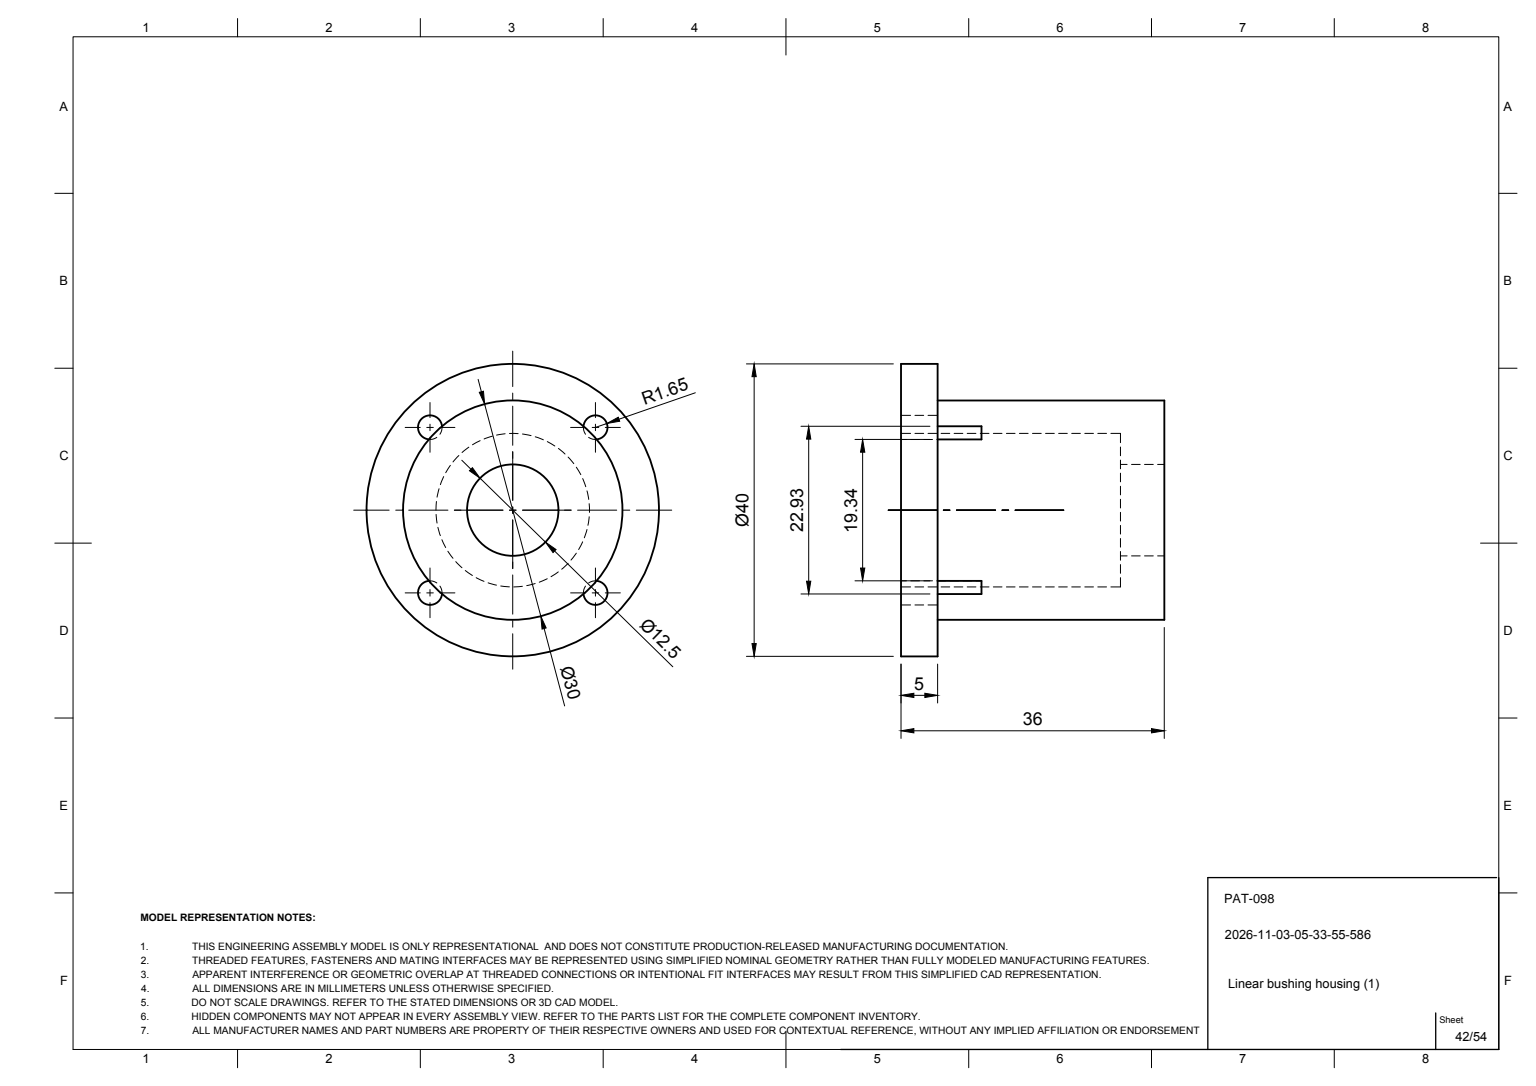
ISO-10303-21;
HEADER;
/* Generated by software containing ST-Developer
 * from STEP Tools, Inc. (www.steptools.com) 
 */

FILE_DESCRIPTION(
/* description */ ('Spring compression tester'),
/* implementation_level */ '2;1');

FILE_NAME(
/* name */ 'Linear bushing housing (1).step',
/* time_stamp */ '2026-10-28T03:24:11-07:00',
/* author */ (''),
/* organization */ (''),
/* preprocessor_version */ 'ST-DEVELOPER v20.2',
/* originating_system */ 'Autodesk Translation Framework v15.17.0.0',
/* authorisation */ '');

FILE_SCHEMA (('AUTOMOTIVE_DESIGN { 1 0 10303 214 3 1 1 }'));
ENDSEC;

DATA;
#10=MECHANICAL_DESIGN_GEOMETRIC_PRESENTATION_REPRESENTATION('',(#1160),#43521);
#1025=SHAPE_REPRESENTATION_RELATIONSHIP('SRR','None',#43840,#1085);
#1085=ADVANCED_BREP_SHAPE_REPRESENTATION('',(#1231),#43500);
#1160=STYLED_ITEM('',(#44181),#1231);
#1231=MANIFOLD_SOLID_BREP('Body1',#18601);
#1521=FACE_BOUND('',#4194,.T.);
#1522=FACE_BOUND('',#4196,.T.);
#1523=FACE_BOUND('',#4200,.T.);
#1524=FACE_BOUND('',#4201,.T.);
#1525=FACE_BOUND('',#4202,.T.);
#1526=FACE_BOUND('',#4203,.T.);
#1527=FACE_BOUND('',#4204,.T.);
#1528=FACE_BOUND('',#4206,.T.);
#2038=PLANE('',#20538);
#2039=PLANE('',#20545);
#2040=PLANE('',#20552);
#2041=PLANE('',#20559);
#2042=PLANE('',#20576);
#2043=PLANE('',#20578);
#2044=PLANE('',#20584);
#2045=PLANE('',#20585);
#2862=FACE_OUTER_BOUND('',#4183,.T.);
#2863=FACE_OUTER_BOUND('',#4184,.T.);
#2864=FACE_OUTER_BOUND('',#4185,.T.);
#2865=FACE_OUTER_BOUND('',#4186,.T.);
#2866=FACE_OUTER_BOUND('',#4187,.T.);
#2867=FACE_OUTER_BOUND('',#4188,.T.);
#2868=FACE_OUTER_BOUND('',#4189,.T.);
#2869=FACE_OUTER_BOUND('',#4190,.T.);
#2870=FACE_OUTER_BOUND('',#4191,.T.);
#2871=FACE_OUTER_BOUND('',#4192,.T.);
#2872=FACE_OUTER_BOUND('',#4193,.T.);
#2873=FACE_OUTER_BOUND('',#4195,.T.);
#2874=FACE_OUTER_BOUND('',#4197,.T.);
#2875=FACE_OUTER_BOUND('',#4198,.T.);
#2876=FACE_OUTER_BOUND('',#4199,.T.);
#2877=FACE_OUTER_BOUND('',#4205,.T.);
#4183=EDGE_LOOP('',(#15357,#15358));
#4184=EDGE_LOOP('',(#15359,#15360,#15361,#15362,#15363,#15364,#15365,#15366));
#4185=EDGE_LOOP('',(#15367,#15368));
#4186=EDGE_LOOP('',(#15369,#15370,#15371,#15372,#15373,#15374,#15375,#15376));
#4187=EDGE_LOOP('',(#15377,#15378,#15379));
#4188=EDGE_LOOP('',(#15380,#15381,#15382,#15383,#15384,#15385,#15386,#15387));
#4189=EDGE_LOOP('',(#15388,#15389,#15390));
#4190=EDGE_LOOP('',(#15391,#15392,#15393,#15394,#15395,#15396,#15397,#15398));
#4191=EDGE_LOOP('',(#15399,#15400,#15401,#15402,#15403,#15404,#15405,#15406,
#15407,#15408,#15409,#15410,#15411,#15412,#15413,#15414,#15415,#15416,#15417,
#15418));
#4192=EDGE_LOOP('',(#15419,#15420,#15421,#15422));
#4193=EDGE_LOOP('',(#15423));
#4194=EDGE_LOOP('',(#15424));
#4195=EDGE_LOOP('',(#15425));
#4196=EDGE_LOOP('',(#15426,#15427,#15428,#15429,#15430,#15431,#15432,#15433,
#15434,#15435,#15436));
#4197=EDGE_LOOP('',(#15437,#15438,#15439,#15440));
#4198=EDGE_LOOP('',(#15441,#15442,#15443,#15444));
#4199=EDGE_LOOP('',(#15445));
#4200=EDGE_LOOP('',(#15446));
#4201=EDGE_LOOP('',(#15447));
#4202=EDGE_LOOP('',(#15448));
#4203=EDGE_LOOP('',(#15449));
#4204=EDGE_LOOP('',(#15450));
#4205=EDGE_LOOP('',(#15451));
#4206=EDGE_LOOP('',(#15452));
#5639=LINE('',#30468,#7071);
#5640=LINE('',#30472,#7072);
#5641=LINE('',#30476,#7073);
#5642=LINE('',#30484,#7074);
#5643=LINE('',#30488,#7075);
#5644=LINE('',#30492,#7076);
#5645=LINE('',#30502,#7077);
#5646=LINE('',#30505,#7078);
#5647=LINE('',#30507,#7079);
#5648=LINE('',#30518,#7080);
#5649=LINE('',#30521,#7081);
#5650=LINE('',#30523,#7082);
#5651=LINE('',#30529,#7083);
#5652=LINE('',#30539,#7084);
#5653=LINE('',#30550,#7085);
#5654=LINE('',#30553,#7086);
#7071=VECTOR('',#24745,1.);
#7072=VECTOR('',#24748,0.165);
#7073=VECTOR('',#24753,1.);
#7074=VECTOR('',#24762,1.);
#7075=VECTOR('',#24765,0.165);
#7076=VECTOR('',#24770,1.);
#7077=VECTOR('',#24781,1.);
#7078=VECTOR('',#24784,1.);
#7079=VECTOR('',#24785,0.165);
#7080=VECTOR('',#24798,1.);
#7081=VECTOR('',#24801,1.);
#7082=VECTOR('',#24802,0.165);
#7083=VECTOR('',#24809,1.5);
#7084=VECTOR('',#24824,1.05);
#7085=VECTOR('',#24839,2.);
#7086=VECTOR('',#24842,0.625);
#7973=CIRCLE('',#20539,1.5);
#7974=CIRCLE('',#20540,0.165);
#7975=CIRCLE('',#20542,0.165);
#7976=CIRCLE('',#20543,0.165);
#7977=CIRCLE('',#20544,0.165);
#7978=CIRCLE('',#20546,1.5);
#7979=CIRCLE('',#20547,0.165);
#7980=CIRCLE('',#20549,0.165);
#7981=CIRCLE('',#20550,0.165);
#7982=CIRCLE('',#20551,0.165);
#7983=CIRCLE('',#20553,1.5);
#7984=CIRCLE('',#20554,0.165);
#7985=CIRCLE('',#20555,0.165);
#7986=CIRCLE('',#20557,0.165);
#7987=CIRCLE('',#20558,0.165);
#7988=CIRCLE('',#20560,1.5);
#7989=CIRCLE('',#20561,0.165);
#7990=CIRCLE('',#20562,0.165);
#7991=CIRCLE('',#20564,0.165);
#7992=CIRCLE('',#20565,0.165);
#7993=CIRCLE('',#20567,1.5);
#7994=CIRCLE('',#20568,1.5);
#7995=CIRCLE('',#20569,1.5);
#7996=CIRCLE('',#20570,1.5);
#7997=CIRCLE('',#20571,1.5);
#7998=CIRCLE('',#20572,1.5);
#7999=CIRCLE('',#20574,1.05);
#8000=CIRCLE('',#20575,1.05);
#8001=CIRCLE('',#20577,0.625);
#8002=CIRCLE('',#20579,2.);
#8003=CIRCLE('',#20581,2.);
#8004=CIRCLE('',#20583,0.625);
#9194=VERTEX_POINT('',#30462);
#9195=VERTEX_POINT('',#30463);
#9196=VERTEX_POINT('',#30467);
#9197=VERTEX_POINT('',#30469);
#9198=VERTEX_POINT('',#30471);
#9199=VERTEX_POINT('',#30474);
#9200=VERTEX_POINT('',#30478);
#9201=VERTEX_POINT('',#30479);
#9202=VERTEX_POINT('',#30483);
#9203=VERTEX_POINT('',#30485);
#9204=VERTEX_POINT('',#30487);
#9205=VERTEX_POINT('',#30490);
#9206=VERTEX_POINT('',#30494);
#9207=VERTEX_POINT('',#30495);
#9208=VERTEX_POINT('',#30497);
#9209=VERTEX_POINT('',#30501);
#9210=VERTEX_POINT('',#30503);
#9211=VERTEX_POINT('',#30506);
#9212=VERTEX_POINT('',#30510);
#9213=VERTEX_POINT('',#30511);
#9214=VERTEX_POINT('',#30513);
#9215=VERTEX_POINT('',#30517);
#9216=VERTEX_POINT('',#30519);
#9217=VERTEX_POINT('',#30522);
#9218=VERTEX_POINT('',#30526);
#9219=VERTEX_POINT('',#30528);
#9220=VERTEX_POINT('',#30536);
#9221=VERTEX_POINT('',#30538);
#9222=VERTEX_POINT('',#30542);
#9223=VERTEX_POINT('',#30545);
#9224=VERTEX_POINT('',#30548);
#9225=VERTEX_POINT('',#30552);
#11343=EDGE_CURVE('',#9194,#9195,#7973,.T.);
#11344=EDGE_CURVE('',#9194,#9195,#7974,.T.);
#11345=EDGE_CURVE('',#9196,#9194,#5639,.T.);
#11346=EDGE_CURVE('',#9197,#9196,#7975,.T.);
#11347=EDGE_CURVE('',#9197,#9198,#5640,.T.);
#11348=EDGE_CURVE('',#9198,#9198,#7976,.T.);
#11349=EDGE_CURVE('',#9199,#9197,#7977,.T.);
#11350=EDGE_CURVE('',#9195,#9199,#5641,.T.);
#11351=EDGE_CURVE('',#9200,#9201,#7978,.T.);
#11352=EDGE_CURVE('',#9200,#9201,#7979,.T.);
#11353=EDGE_CURVE('',#9202,#9200,#5642,.T.);
#11354=EDGE_CURVE('',#9203,#9202,#7980,.T.);
#11355=EDGE_CURVE('',#9203,#9204,#5643,.T.);
#11356=EDGE_CURVE('',#9204,#9204,#7981,.T.);
#11357=EDGE_CURVE('',#9205,#9203,#7982,.T.);
#11358=EDGE_CURVE('',#9201,#9205,#5644,.T.);
#11359=EDGE_CURVE('',#9206,#9207,#7983,.T.);
#11360=EDGE_CURVE('',#9206,#9208,#7984,.T.);
#11361=EDGE_CURVE('',#9208,#9207,#7985,.T.);
#11362=EDGE_CURVE('',#9209,#9206,#5645,.T.);
#11363=EDGE_CURVE('',#9210,#9209,#7986,.T.);
#11364=EDGE_CURVE('',#9207,#9210,#5646,.T.);
#11365=EDGE_CURVE('',#9208,#9211,#5647,.T.);
#11366=EDGE_CURVE('',#9211,#9211,#7987,.T.);
#11367=EDGE_CURVE('',#9212,#9213,#7988,.T.);
#11368=EDGE_CURVE('',#9212,#9214,#7989,.T.);
#11369=EDGE_CURVE('',#9214,#9213,#7990,.T.);
#11370=EDGE_CURVE('',#9215,#9212,#5648,.T.);
#11371=EDGE_CURVE('',#9216,#9215,#7991,.T.);
#11372=EDGE_CURVE('',#9213,#9216,#5649,.T.);
#11373=EDGE_CURVE('',#9214,#9217,#5650,.T.);
#11374=EDGE_CURVE('',#9217,#9217,#7992,.T.);
#11375=EDGE_CURVE('',#9199,#9218,#7993,.T.);
#11376=EDGE_CURVE('',#9218,#9219,#5651,.T.);
#11377=EDGE_CURVE('',#9219,#9219,#7994,.T.);
#11378=EDGE_CURVE('',#9218,#9202,#7995,.T.);
#11379=EDGE_CURVE('',#9205,#9209,#7996,.T.);
#11380=EDGE_CURVE('',#9210,#9215,#7997,.T.);
#11381=EDGE_CURVE('',#9216,#9196,#7998,.T.);
#11382=EDGE_CURVE('',#9220,#9220,#7999,.T.);
#11383=EDGE_CURVE('',#9220,#9221,#5652,.T.);
#11384=EDGE_CURVE('',#9221,#9221,#8000,.T.);
#11385=EDGE_CURVE('',#9222,#9222,#8001,.T.);
#11386=EDGE_CURVE('',#9223,#9223,#8002,.T.);
#11387=EDGE_CURVE('',#9224,#9224,#8003,.T.);
#11388=EDGE_CURVE('',#9224,#9223,#5653,.T.);
#11389=EDGE_CURVE('',#9222,#9225,#5654,.T.);
#11390=EDGE_CURVE('',#9225,#9225,#8004,.T.);
#15357=ORIENTED_EDGE('',*,*,#11343,.F.);
#15358=ORIENTED_EDGE('',*,*,#11344,.T.);
#15359=ORIENTED_EDGE('',*,*,#11345,.F.);
#15360=ORIENTED_EDGE('',*,*,#11346,.F.);
#15361=ORIENTED_EDGE('',*,*,#11347,.T.);
#15362=ORIENTED_EDGE('',*,*,#11348,.F.);
#15363=ORIENTED_EDGE('',*,*,#11347,.F.);
#15364=ORIENTED_EDGE('',*,*,#11349,.F.);
#15365=ORIENTED_EDGE('',*,*,#11350,.F.);
#15366=ORIENTED_EDGE('',*,*,#11344,.F.);
#15367=ORIENTED_EDGE('',*,*,#11351,.F.);
#15368=ORIENTED_EDGE('',*,*,#11352,.T.);
#15369=ORIENTED_EDGE('',*,*,#11353,.F.);
#15370=ORIENTED_EDGE('',*,*,#11354,.F.);
#15371=ORIENTED_EDGE('',*,*,#11355,.T.);
#15372=ORIENTED_EDGE('',*,*,#11356,.F.);
#15373=ORIENTED_EDGE('',*,*,#11355,.F.);
#15374=ORIENTED_EDGE('',*,*,#11357,.F.);
#15375=ORIENTED_EDGE('',*,*,#11358,.F.);
#15376=ORIENTED_EDGE('',*,*,#11352,.F.);
#15377=ORIENTED_EDGE('',*,*,#11359,.F.);
#15378=ORIENTED_EDGE('',*,*,#11360,.T.);
#15379=ORIENTED_EDGE('',*,*,#11361,.T.);
#15380=ORIENTED_EDGE('',*,*,#11362,.F.);
#15381=ORIENTED_EDGE('',*,*,#11363,.F.);
#15382=ORIENTED_EDGE('',*,*,#11364,.F.);
#15383=ORIENTED_EDGE('',*,*,#11361,.F.);
#15384=ORIENTED_EDGE('',*,*,#11365,.T.);
#15385=ORIENTED_EDGE('',*,*,#11366,.F.);
#15386=ORIENTED_EDGE('',*,*,#11365,.F.);
#15387=ORIENTED_EDGE('',*,*,#11360,.F.);
#15388=ORIENTED_EDGE('',*,*,#11367,.F.);
#15389=ORIENTED_EDGE('',*,*,#11368,.T.);
#15390=ORIENTED_EDGE('',*,*,#11369,.T.);
#15391=ORIENTED_EDGE('',*,*,#11370,.F.);
#15392=ORIENTED_EDGE('',*,*,#11371,.F.);
#15393=ORIENTED_EDGE('',*,*,#11372,.F.);
#15394=ORIENTED_EDGE('',*,*,#11369,.F.);
#15395=ORIENTED_EDGE('',*,*,#11373,.T.);
#15396=ORIENTED_EDGE('',*,*,#11374,.F.);
#15397=ORIENTED_EDGE('',*,*,#11373,.F.);
#15398=ORIENTED_EDGE('',*,*,#11368,.F.);
#15399=ORIENTED_EDGE('',*,*,#11345,.T.);
#15400=ORIENTED_EDGE('',*,*,#11343,.T.);
#15401=ORIENTED_EDGE('',*,*,#11350,.T.);
#15402=ORIENTED_EDGE('',*,*,#11375,.T.);
#15403=ORIENTED_EDGE('',*,*,#11376,.T.);
#15404=ORIENTED_EDGE('',*,*,#11377,.T.);
#15405=ORIENTED_EDGE('',*,*,#11376,.F.);
#15406=ORIENTED_EDGE('',*,*,#11378,.T.);
#15407=ORIENTED_EDGE('',*,*,#11353,.T.);
#15408=ORIENTED_EDGE('',*,*,#11351,.T.);
#15409=ORIENTED_EDGE('',*,*,#11358,.T.);
#15410=ORIENTED_EDGE('',*,*,#11379,.T.);
#15411=ORIENTED_EDGE('',*,*,#11362,.T.);
#15412=ORIENTED_EDGE('',*,*,#11359,.T.);
#15413=ORIENTED_EDGE('',*,*,#11364,.T.);
#15414=ORIENTED_EDGE('',*,*,#11380,.T.);
#15415=ORIENTED_EDGE('',*,*,#11370,.T.);
#15416=ORIENTED_EDGE('',*,*,#11367,.T.);
#15417=ORIENTED_EDGE('',*,*,#11372,.T.);
#15418=ORIENTED_EDGE('',*,*,#11381,.T.);
#15419=ORIENTED_EDGE('',*,*,#11382,.F.);
#15420=ORIENTED_EDGE('',*,*,#11383,.T.);
#15421=ORIENTED_EDGE('',*,*,#11384,.F.);
#15422=ORIENTED_EDGE('',*,*,#11383,.F.);
#15423=ORIENTED_EDGE('',*,*,#11382,.T.);
#15424=ORIENTED_EDGE('',*,*,#11385,.F.);
#15425=ORIENTED_EDGE('',*,*,#11386,.F.);
#15426=ORIENTED_EDGE('',*,*,#11349,.T.);
#15427=ORIENTED_EDGE('',*,*,#11346,.T.);
#15428=ORIENTED_EDGE('',*,*,#11381,.F.);
#15429=ORIENTED_EDGE('',*,*,#11371,.T.);
#15430=ORIENTED_EDGE('',*,*,#11380,.F.);
#15431=ORIENTED_EDGE('',*,*,#11363,.T.);
#15432=ORIENTED_EDGE('',*,*,#11379,.F.);
#15433=ORIENTED_EDGE('',*,*,#11357,.T.);
#15434=ORIENTED_EDGE('',*,*,#11354,.T.);
#15435=ORIENTED_EDGE('',*,*,#11378,.F.);
#15436=ORIENTED_EDGE('',*,*,#11375,.F.);
#15437=ORIENTED_EDGE('',*,*,#11387,.F.);
#15438=ORIENTED_EDGE('',*,*,#11388,.T.);
#15439=ORIENTED_EDGE('',*,*,#11386,.T.);
#15440=ORIENTED_EDGE('',*,*,#11388,.F.);
#15441=ORIENTED_EDGE('',*,*,#11385,.T.);
#15442=ORIENTED_EDGE('',*,*,#11389,.T.);
#15443=ORIENTED_EDGE('',*,*,#11390,.T.);
#15444=ORIENTED_EDGE('',*,*,#11389,.F.);
#15445=ORIENTED_EDGE('',*,*,#11387,.T.);
#15446=ORIENTED_EDGE('',*,*,#11384,.T.);
#15447=ORIENTED_EDGE('',*,*,#11374,.T.);
#15448=ORIENTED_EDGE('',*,*,#11366,.T.);
#15449=ORIENTED_EDGE('',*,*,#11356,.T.);
#15450=ORIENTED_EDGE('',*,*,#11348,.T.);
#15451=ORIENTED_EDGE('',*,*,#11377,.F.);
#15452=ORIENTED_EDGE('',*,*,#11390,.F.);
#17288=CYLINDRICAL_SURFACE('',#20541,0.165);
#17289=CYLINDRICAL_SURFACE('',#20548,0.165);
#17290=CYLINDRICAL_SURFACE('',#20556,0.165);
#17291=CYLINDRICAL_SURFACE('',#20563,0.165);
#17292=CYLINDRICAL_SURFACE('',#20566,1.5);
#17293=CYLINDRICAL_SURFACE('',#20573,1.05);
#17294=CYLINDRICAL_SURFACE('',#20580,2.);
#17295=CYLINDRICAL_SURFACE('',#20582,0.625);
#18186=ADVANCED_FACE('',(#2862),#2038,.T.);
#18187=ADVANCED_FACE('',(#2863),#17288,.F.);
#18188=ADVANCED_FACE('',(#2864),#2039,.T.);
#18189=ADVANCED_FACE('',(#2865),#17289,.F.);
#18190=ADVANCED_FACE('',(#2866),#2040,.T.);
#18191=ADVANCED_FACE('',(#2867),#17290,.F.);
#18192=ADVANCED_FACE('',(#2868),#2041,.T.);
#18193=ADVANCED_FACE('',(#2869),#17291,.F.);
#18194=ADVANCED_FACE('',(#2870),#17292,.T.);
#18195=ADVANCED_FACE('',(#2871),#17293,.F.);
#18196=ADVANCED_FACE('',(#2872,#1521),#2042,.T.);
#18197=ADVANCED_FACE('',(#2873,#1522),#2043,.F.);
#18198=ADVANCED_FACE('',(#2874),#17294,.T.);
#18199=ADVANCED_FACE('',(#2875),#17295,.F.);
#18200=ADVANCED_FACE('',(#2876,#1523,#1524,#1525,#1526,#1527),#2044,.T.);
#18201=ADVANCED_FACE('',(#2877,#1528),#2045,.F.);
#18601=CLOSED_SHELL('',(#18186,#18187,#18188,#18189,#18190,#18191,#18192,
#18193,#18194,#18195,#18196,#18197,#18198,#18199,#18200,#18201));
#20537=AXIS2_PLACEMENT_3D('',#30460,#24735,#24736);
#20538=AXIS2_PLACEMENT_3D('',#30461,#24737,#24738);
#20539=AXIS2_PLACEMENT_3D('',#30464,#24739,#24740);
#20540=AXIS2_PLACEMENT_3D('',#30465,#24741,#24742);
#20541=AXIS2_PLACEMENT_3D('',#30466,#24743,#24744);
#20542=AXIS2_PLACEMENT_3D('',#30470,#24746,#24747);
#20543=AXIS2_PLACEMENT_3D('',#30473,#24749,#24750);
#20544=AXIS2_PLACEMENT_3D('',#30475,#24751,#24752);
#20545=AXIS2_PLACEMENT_3D('',#30477,#24754,#24755);
#20546=AXIS2_PLACEMENT_3D('',#30480,#24756,#24757);
#20547=AXIS2_PLACEMENT_3D('',#30481,#24758,#24759);
#20548=AXIS2_PLACEMENT_3D('',#30482,#24760,#24761);
#20549=AXIS2_PLACEMENT_3D('',#30486,#24763,#24764);
#20550=AXIS2_PLACEMENT_3D('',#30489,#24766,#24767);
#20551=AXIS2_PLACEMENT_3D('',#30491,#24768,#24769);
#20552=AXIS2_PLACEMENT_3D('',#30493,#24771,#24772);
#20553=AXIS2_PLACEMENT_3D('',#30496,#24773,#24774);
#20554=AXIS2_PLACEMENT_3D('',#30498,#24775,#24776);
#20555=AXIS2_PLACEMENT_3D('',#30499,#24777,#24778);
#20556=AXIS2_PLACEMENT_3D('',#30500,#24779,#24780);
#20557=AXIS2_PLACEMENT_3D('',#30504,#24782,#24783);
#20558=AXIS2_PLACEMENT_3D('',#30508,#24786,#24787);
#20559=AXIS2_PLACEMENT_3D('',#30509,#24788,#24789);
#20560=AXIS2_PLACEMENT_3D('',#30512,#24790,#24791);
#20561=AXIS2_PLACEMENT_3D('',#30514,#24792,#24793);
#20562=AXIS2_PLACEMENT_3D('',#30515,#24794,#24795);
#20563=AXIS2_PLACEMENT_3D('',#30516,#24796,#24797);
#20564=AXIS2_PLACEMENT_3D('',#30520,#24799,#24800);
#20565=AXIS2_PLACEMENT_3D('',#30524,#24803,#24804);
#20566=AXIS2_PLACEMENT_3D('',#30525,#24805,#24806);
#20567=AXIS2_PLACEMENT_3D('',#30527,#24807,#24808);
#20568=AXIS2_PLACEMENT_3D('',#30530,#24810,#24811);
#20569=AXIS2_PLACEMENT_3D('',#30531,#24812,#24813);
#20570=AXIS2_PLACEMENT_3D('',#30532,#24814,#24815);
#20571=AXIS2_PLACEMENT_3D('',#30533,#24816,#24817);
#20572=AXIS2_PLACEMENT_3D('',#30534,#24818,#24819);
#20573=AXIS2_PLACEMENT_3D('',#30535,#24820,#24821);
#20574=AXIS2_PLACEMENT_3D('',#30537,#24822,#24823);
#20575=AXIS2_PLACEMENT_3D('',#30540,#24825,#24826);
#20576=AXIS2_PLACEMENT_3D('',#30541,#24827,#24828);
#20577=AXIS2_PLACEMENT_3D('',#30543,#24829,#24830);
#20578=AXIS2_PLACEMENT_3D('',#30544,#24831,#24832);
#20579=AXIS2_PLACEMENT_3D('',#30546,#24833,#24834);
#20580=AXIS2_PLACEMENT_3D('',#30547,#24835,#24836);
#20581=AXIS2_PLACEMENT_3D('',#30549,#24837,#24838);
#20582=AXIS2_PLACEMENT_3D('',#30551,#24840,#24841);
#20583=AXIS2_PLACEMENT_3D('',#30554,#24843,#24844);
#20584=AXIS2_PLACEMENT_3D('',#30555,#24845,#24846);
#20585=AXIS2_PLACEMENT_3D('',#30556,#24847,#24848);
#24735=DIRECTION('axis',(0.,0.,1.));
#24736=DIRECTION('refdir',(1.,0.,0.));
#24737=DIRECTION('center_axis',(0.,0.,1.));
#24738=DIRECTION('ref_axis',(1.,0.,0.));
#24739=DIRECTION('center_axis',(0.,0.,-1.));
#24740=DIRECTION('ref_axis',(1.,0.,0.));
#24741=DIRECTION('center_axis',(0.,0.,1.));
#24742=DIRECTION('ref_axis',(1.,0.,0.));
#24743=DIRECTION('center_axis',(0.,0.,1.));
#24744=DIRECTION('ref_axis',(1.,0.,0.));
#24745=DIRECTION('',(0.,0.,-1.));
#24746=DIRECTION('center_axis',(0.,0.,1.));
#24747=DIRECTION('ref_axis',(1.,0.,0.));
#24748=DIRECTION('',(0.,0.,1.));
#24749=DIRECTION('center_axis',(0.,0.,-1.));
#24750=DIRECTION('ref_axis',(1.,0.,0.));
#24751=DIRECTION('center_axis',(0.,0.,1.));
#24752=DIRECTION('ref_axis',(1.,0.,0.));
#24753=DIRECTION('',(0.,0.,1.));
#24754=DIRECTION('center_axis',(0.,0.,1.));
#24755=DIRECTION('ref_axis',(1.,0.,0.));
#24756=DIRECTION('center_axis',(0.,0.,-1.));
#24757=DIRECTION('ref_axis',(1.,0.,0.));
#24758=DIRECTION('center_axis',(0.,0.,1.));
#24759=DIRECTION('ref_axis',(1.,0.,0.));
#24760=DIRECTION('center_axis',(0.,0.,1.));
#24761=DIRECTION('ref_axis',(1.,0.,0.));
#24762=DIRECTION('',(0.,0.,-1.));
#24763=DIRECTION('center_axis',(0.,0.,1.));
#24764=DIRECTION('ref_axis',(1.,0.,0.));
#24765=DIRECTION('',(0.,0.,1.));
#24766=DIRECTION('center_axis',(0.,0.,-1.));
#24767=DIRECTION('ref_axis',(1.,0.,0.));
#24768=DIRECTION('center_axis',(0.,0.,1.));
#24769=DIRECTION('ref_axis',(1.,0.,0.));
#24770=DIRECTION('',(0.,0.,1.));
#24771=DIRECTION('center_axis',(0.,0.,1.));
#24772=DIRECTION('ref_axis',(1.,0.,0.));
#24773=DIRECTION('center_axis',(0.,0.,-1.));
#24774=DIRECTION('ref_axis',(1.,0.,0.));
#24775=DIRECTION('center_axis',(0.,0.,1.));
#24776=DIRECTION('ref_axis',(1.,0.,0.));
#24777=DIRECTION('center_axis',(0.,0.,1.));
#24778=DIRECTION('ref_axis',(1.,0.,0.));
#24779=DIRECTION('center_axis',(0.,0.,1.));
#24780=DIRECTION('ref_axis',(1.,0.,0.));
#24781=DIRECTION('',(0.,0.,-1.));
#24782=DIRECTION('center_axis',(0.,0.,1.));
#24783=DIRECTION('ref_axis',(1.,0.,0.));
#24784=DIRECTION('',(0.,0.,1.));
#24785=DIRECTION('',(0.,0.,1.));
#24786=DIRECTION('center_axis',(0.,0.,-1.));
#24787=DIRECTION('ref_axis',(1.,0.,0.));
#24788=DIRECTION('center_axis',(0.,0.,1.));
#24789=DIRECTION('ref_axis',(1.,0.,0.));
#24790=DIRECTION('center_axis',(0.,0.,-1.));
#24791=DIRECTION('ref_axis',(1.,0.,0.));
#24792=DIRECTION('center_axis',(0.,0.,1.));
#24793=DIRECTION('ref_axis',(1.,0.,0.));
#24794=DIRECTION('center_axis',(0.,0.,1.));
#24795=DIRECTION('ref_axis',(1.,0.,0.));
#24796=DIRECTION('center_axis',(0.,0.,1.));
#24797=DIRECTION('ref_axis',(1.,0.,0.));
#24798=DIRECTION('',(0.,0.,-1.));
#24799=DIRECTION('center_axis',(0.,0.,1.));
#24800=DIRECTION('ref_axis',(1.,0.,0.));
#24801=DIRECTION('',(0.,0.,1.));
#24802=DIRECTION('',(0.,0.,1.));
#24803=DIRECTION('center_axis',(0.,0.,-1.));
#24804=DIRECTION('ref_axis',(1.,0.,0.));
#24805=DIRECTION('center_axis',(0.,0.,1.));
#24806=DIRECTION('ref_axis',(1.,0.,0.));
#24807=DIRECTION('center_axis',(0.,0.,-1.));
#24808=DIRECTION('ref_axis',(1.,0.,0.));
#24809=DIRECTION('',(0.,0.,-1.));
#24810=DIRECTION('center_axis',(0.,0.,1.));
#24811=DIRECTION('ref_axis',(1.,0.,0.));
#24812=DIRECTION('center_axis',(0.,0.,-1.));
#24813=DIRECTION('ref_axis',(1.,0.,0.));
#24814=DIRECTION('center_axis',(0.,0.,-1.));
#24815=DIRECTION('ref_axis',(1.,0.,0.));
#24816=DIRECTION('center_axis',(0.,0.,-1.));
#24817=DIRECTION('ref_axis',(1.,0.,0.));
#24818=DIRECTION('center_axis',(0.,0.,-1.));
#24819=DIRECTION('ref_axis',(1.,0.,0.));
#24820=DIRECTION('center_axis',(0.,0.,1.));
#24821=DIRECTION('ref_axis',(1.,0.,0.));
#24822=DIRECTION('center_axis',(0.,0.,1.));
#24823=DIRECTION('ref_axis',(1.,0.,0.));
#24824=DIRECTION('',(0.,0.,1.));
#24825=DIRECTION('center_axis',(0.,0.,-1.));
#24826=DIRECTION('ref_axis',(1.,0.,0.));
#24827=DIRECTION('center_axis',(0.,0.,1.));
#24828=DIRECTION('ref_axis',(1.,0.,0.));
#24829=DIRECTION('center_axis',(0.,0.,1.));
#24830=DIRECTION('ref_axis',(1.,0.,0.));
#24831=DIRECTION('center_axis',(0.,0.,1.));
#24832=DIRECTION('ref_axis',(1.,0.,0.));
#24833=DIRECTION('center_axis',(0.,0.,1.));
#24834=DIRECTION('ref_axis',(1.,0.,0.));
#24835=DIRECTION('center_axis',(0.,0.,1.));
#24836=DIRECTION('ref_axis',(1.,0.,0.));
#24837=DIRECTION('center_axis',(0.,0.,1.));
#24838=DIRECTION('ref_axis',(1.,0.,0.));
#24839=DIRECTION('',(0.,0.,-1.));
#24840=DIRECTION('center_axis',(0.,0.,1.));
#24841=DIRECTION('ref_axis',(1.,0.,0.));
#24842=DIRECTION('',(0.,0.,-1.));
#24843=DIRECTION('center_axis',(0.,0.,-1.));
#24844=DIRECTION('ref_axis',(1.,0.,0.));
#24845=DIRECTION('center_axis',(0.,0.,1.));
#24846=DIRECTION('ref_axis',(1.,0.,0.));
#24847=DIRECTION('center_axis',(0.,0.,1.));
#24848=DIRECTION('ref_axis',(1.,0.,0.));
#30460=CARTESIAN_POINT('',(0.,0.,0.));
#30461=CARTESIAN_POINT('Origin',(4.86862915010152,-1.13137084989848,14.));
#30462=CARTESIAN_POINT('',(5.03292205834015,-1.14662995545858,14.));
#30463=CARTESIAN_POINT('',(4.85337004454142,-0.96707794165985,14.));
#30464=CARTESIAN_POINT('Origin',(6.,0.,14.));
#30465=CARTESIAN_POINT('Origin',(4.86862915010152,-1.13137084989848,14.));
#30466=CARTESIAN_POINT('Origin',(4.86862915010152,-1.13137084989848,14.));
#30467=CARTESIAN_POINT('',(5.03292205834015,-1.14662995545858,14.6));
#30468=CARTESIAN_POINT('',(5.03292205834015,-1.14662995545858,14.));
#30469=CARTESIAN_POINT('',(4.70362915010152,-1.13137084989848,14.6));
#30470=CARTESIAN_POINT('Origin',(4.86862915010152,-1.13137084989848,14.6));
#30471=CARTESIAN_POINT('',(4.70362915010152,-1.13137084989848,15.1));
#30472=CARTESIAN_POINT('',(4.70362915010152,-1.13137084989848,14.));
#30473=CARTESIAN_POINT('Origin',(4.86862915010152,-1.13137084989848,15.1));
#30474=CARTESIAN_POINT('',(4.85337004454142,-0.967077941659851,14.6));
#30475=CARTESIAN_POINT('Origin',(4.86862915010152,-1.13137084989848,14.6));
#30476=CARTESIAN_POINT('',(4.85337004454142,-0.96707794165985,14.));
#30477=CARTESIAN_POINT('Origin',(4.86862915010152,1.13137084989848,14.));
#30478=CARTESIAN_POINT('',(4.85337004454142,0.96707794165985,14.));
#30479=CARTESIAN_POINT('',(5.03292205834015,1.14662995545858,14.));
#30480=CARTESIAN_POINT('Origin',(6.,0.,14.));
#30481=CARTESIAN_POINT('Origin',(4.86862915010152,1.13137084989848,14.));
#30482=CARTESIAN_POINT('Origin',(4.86862915010152,1.13137084989848,14.));
#30483=CARTESIAN_POINT('',(4.85337004454142,0.967077941659849,14.6));
#30484=CARTESIAN_POINT('',(4.85337004454142,0.96707794165985,14.));
#30485=CARTESIAN_POINT('',(4.70362915010152,1.13137084989848,14.6));
#30486=CARTESIAN_POINT('Origin',(4.86862915010152,1.13137084989848,14.6));
#30487=CARTESIAN_POINT('',(4.70362915010152,1.13137084989848,15.1));
#30488=CARTESIAN_POINT('',(4.70362915010152,1.13137084989848,14.));
#30489=CARTESIAN_POINT('Origin',(4.86862915010152,1.13137084989848,15.1));
#30490=CARTESIAN_POINT('',(5.03292205834015,1.14662995545858,14.6));
#30491=CARTESIAN_POINT('Origin',(4.86862915010152,1.13137084989848,14.6));
#30492=CARTESIAN_POINT('',(5.03292205834015,1.14662995545858,14.));
#30493=CARTESIAN_POINT('Origin',(7.13137084989848,1.13137084989848,14.));
#30494=CARTESIAN_POINT('',(6.96707794165985,1.14662995545858,14.));
#30495=CARTESIAN_POINT('',(7.14662995545858,0.96707794165985,14.));
#30496=CARTESIAN_POINT('Origin',(6.,0.,14.));
#30497=CARTESIAN_POINT('',(6.96637084989848,1.13137084989848,14.));
#30498=CARTESIAN_POINT('Origin',(7.13137084989848,1.13137084989848,14.));
#30499=CARTESIAN_POINT('Origin',(7.13137084989848,1.13137084989848,14.));
#30500=CARTESIAN_POINT('Origin',(7.13137084989848,1.13137084989848,14.));
#30501=CARTESIAN_POINT('',(6.96707794165985,1.14662995545858,14.6));
#30502=CARTESIAN_POINT('',(6.96707794165985,1.14662995545858,14.));
#30503=CARTESIAN_POINT('',(7.14662995545858,0.967077941659851,14.6));
#30504=CARTESIAN_POINT('Origin',(7.13137084989848,1.13137084989848,14.6));
#30505=CARTESIAN_POINT('',(7.14662995545858,0.96707794165985,14.));
#30506=CARTESIAN_POINT('',(6.96637084989848,1.13137084989848,15.1));
#30507=CARTESIAN_POINT('',(6.96637084989848,1.13137084989848,14.));
#30508=CARTESIAN_POINT('Origin',(7.13137084989848,1.13137084989848,15.1));
#30509=CARTESIAN_POINT('Origin',(7.13137084989848,-1.13137084989848,14.));
#30510=CARTESIAN_POINT('',(7.14662995545858,-0.96707794165985,14.));
#30511=CARTESIAN_POINT('',(6.96707794165985,-1.14662995545858,14.));
#30512=CARTESIAN_POINT('Origin',(6.,0.,14.));
#30513=CARTESIAN_POINT('',(6.96637084989848,-1.13137084989848,14.));
#30514=CARTESIAN_POINT('Origin',(7.13137084989848,-1.13137084989848,14.));
#30515=CARTESIAN_POINT('Origin',(7.13137084989848,-1.13137084989848,14.));
#30516=CARTESIAN_POINT('Origin',(7.13137084989848,-1.13137084989848,14.));
#30517=CARTESIAN_POINT('',(7.14662995545858,-0.967077941659849,14.6));
#30518=CARTESIAN_POINT('',(7.14662995545858,-0.96707794165985,14.));
#30519=CARTESIAN_POINT('',(6.96707794165985,-1.14662995545858,14.6));
#30520=CARTESIAN_POINT('Origin',(7.13137084989848,-1.13137084989848,14.6));
#30521=CARTESIAN_POINT('',(6.96707794165985,-1.14662995545858,14.));
#30522=CARTESIAN_POINT('',(6.96637084989848,-1.13137084989848,15.1));
#30523=CARTESIAN_POINT('',(6.96637084989848,-1.13137084989848,14.));
#30524=CARTESIAN_POINT('Origin',(7.13137084989848,-1.13137084989848,15.1));
#30525=CARTESIAN_POINT('Origin',(6.,0.,11.5));
#30526=CARTESIAN_POINT('',(4.5,-1.83697019872103E-16,14.6));
#30527=CARTESIAN_POINT('Origin',(6.,0.,14.6));
#30528=CARTESIAN_POINT('',(4.5,-1.83697019872103E-16,11.5));
#30529=CARTESIAN_POINT('',(4.5,-1.83697019872103E-16,11.5));
#30530=CARTESIAN_POINT('Origin',(6.,0.,11.5));
#30531=CARTESIAN_POINT('Origin',(6.,0.,14.6));
#30532=CARTESIAN_POINT('Origin',(6.,0.,14.6));
#30533=CARTESIAN_POINT('Origin',(6.,0.,14.6));
#30534=CARTESIAN_POINT('Origin',(6.,0.,14.6));
#30535=CARTESIAN_POINT('Origin',(6.,0.,12.1));
#30536=CARTESIAN_POINT('',(4.95,-1.28587913910472E-16,12.1));
#30537=CARTESIAN_POINT('Origin',(6.,0.,12.1));
#30538=CARTESIAN_POINT('',(4.95,1.28587913910472E-16,15.1));
#30539=CARTESIAN_POINT('',(4.95,-1.28587913910472E-16,12.1));
#30540=CARTESIAN_POINT('Origin',(6.,0.,15.1));
#30541=CARTESIAN_POINT('Origin',(6.,0.,12.1));
#30542=CARTESIAN_POINT('',(5.375,-7.65404249467096E-17,12.1));
#30543=CARTESIAN_POINT('Origin',(6.,0.,12.1));
#30544=CARTESIAN_POINT('Origin',(6.,0.,14.6));
#30545=CARTESIAN_POINT('',(4.,-2.44929359829471E-16,14.6));
#30546=CARTESIAN_POINT('Origin',(6.,0.,14.6));
#30547=CARTESIAN_POINT('Origin',(6.,0.,14.6));
#30548=CARTESIAN_POINT('',(4.,-2.44929359829471E-16,15.1));
#30549=CARTESIAN_POINT('Origin',(6.,0.,15.1));
#30550=CARTESIAN_POINT('',(4.,-2.44929359829471E-16,14.6));
#30551=CARTESIAN_POINT('Origin',(6.,0.,11.5));
#30552=CARTESIAN_POINT('',(5.375,-7.65404249467096E-17,11.5));
#30553=CARTESIAN_POINT('',(5.375,-7.65404249467096E-17,11.5));
#30554=CARTESIAN_POINT('Origin',(6.,0.,11.5));
#30555=CARTESIAN_POINT('Origin',(6.,0.,15.1));
#30556=CARTESIAN_POINT('Origin',(6.,0.,11.5));
#43432=UNCERTAINTY_MEASURE_WITH_UNIT(LENGTH_MEASURE(0.001),#43522,
'DISTANCE_ACCURACY_VALUE',
'Maximum model space distance between geometric entities at asserted c
onnectivities');
#43453=UNCERTAINTY_MEASURE_WITH_UNIT(LENGTH_MEASURE(0.001),#43522,
'DISTANCE_ACCURACY_VALUE',
'Maximum model space distance between geometric entities at asserted c
onnectivities');
#43500=(
GEOMETRIC_REPRESENTATION_CONTEXT(3)
GLOBAL_UNCERTAINTY_ASSIGNED_CONTEXT((#43432))
GLOBAL_UNIT_ASSIGNED_CONTEXT((#43522,#43524,#43525))
REPRESENTATION_CONTEXT('','3D')
);
#43521=(
GEOMETRIC_REPRESENTATION_CONTEXT(3)
GLOBAL_UNCERTAINTY_ASSIGNED_CONTEXT((#43453))
GLOBAL_UNIT_ASSIGNED_CONTEXT((#43522,#43524,#43525))
REPRESENTATION_CONTEXT('','3D')
);
#43522=(
LENGTH_UNIT()
NAMED_UNIT(*)
SI_UNIT(.CENTI.,.METRE.)
);
#43524=(
NAMED_UNIT(*)
PLANE_ANGLE_UNIT()
SI_UNIT($,.RADIAN.)
);
#43525=(
NAMED_UNIT(*)
SI_UNIT($,.STERADIAN.)
SOLID_ANGLE_UNIT()
);
#43572=SHAPE_DEFINITION_REPRESENTATION(#43649,#43840);
#43649=PRODUCT_DEFINITION_SHAPE('',$,#43908);
#43840=SHAPE_REPRESENTATION('',(#20537),#43500);
#43861=PRODUCT_DEFINITION_CONTEXT('part definition',#44064,'design');
#43908=PRODUCT_DEFINITION('Linear bushing housing (1)',
'Linear bushing housing (1)',#43975,#43861);
#43975=PRODUCT_DEFINITION_FORMATION('',$,#44112);
#44064=APPLICATION_CONTEXT(
'Core Data for Automotive Mechanical Design Process');
#44065=PRODUCT_CONTEXT('part definition',#44064,'mechanical');
#44112=PRODUCT('Linear bushing housing (1)','Linear bushing housing (1)',
'Linear bushing housing (1)',(#44065));
#44175=COLOUR_RGB('Dark Blue',0.08,0.2,0.34);
#44176=FILL_AREA_STYLE_COLOUR('',#44175);
#44177=FILL_AREA_STYLE('',(#44176));
#44178=SURFACE_STYLE_FILL_AREA(#44177);
#44179=SURFACE_SIDE_STYLE('',(#44178));
#44180=SURFACE_STYLE_USAGE(.BOTH.,#44179);
#44181=PRESENTATION_STYLE_ASSIGNMENT((#44180));
ENDSEC;
END-ISO-10303-21;
